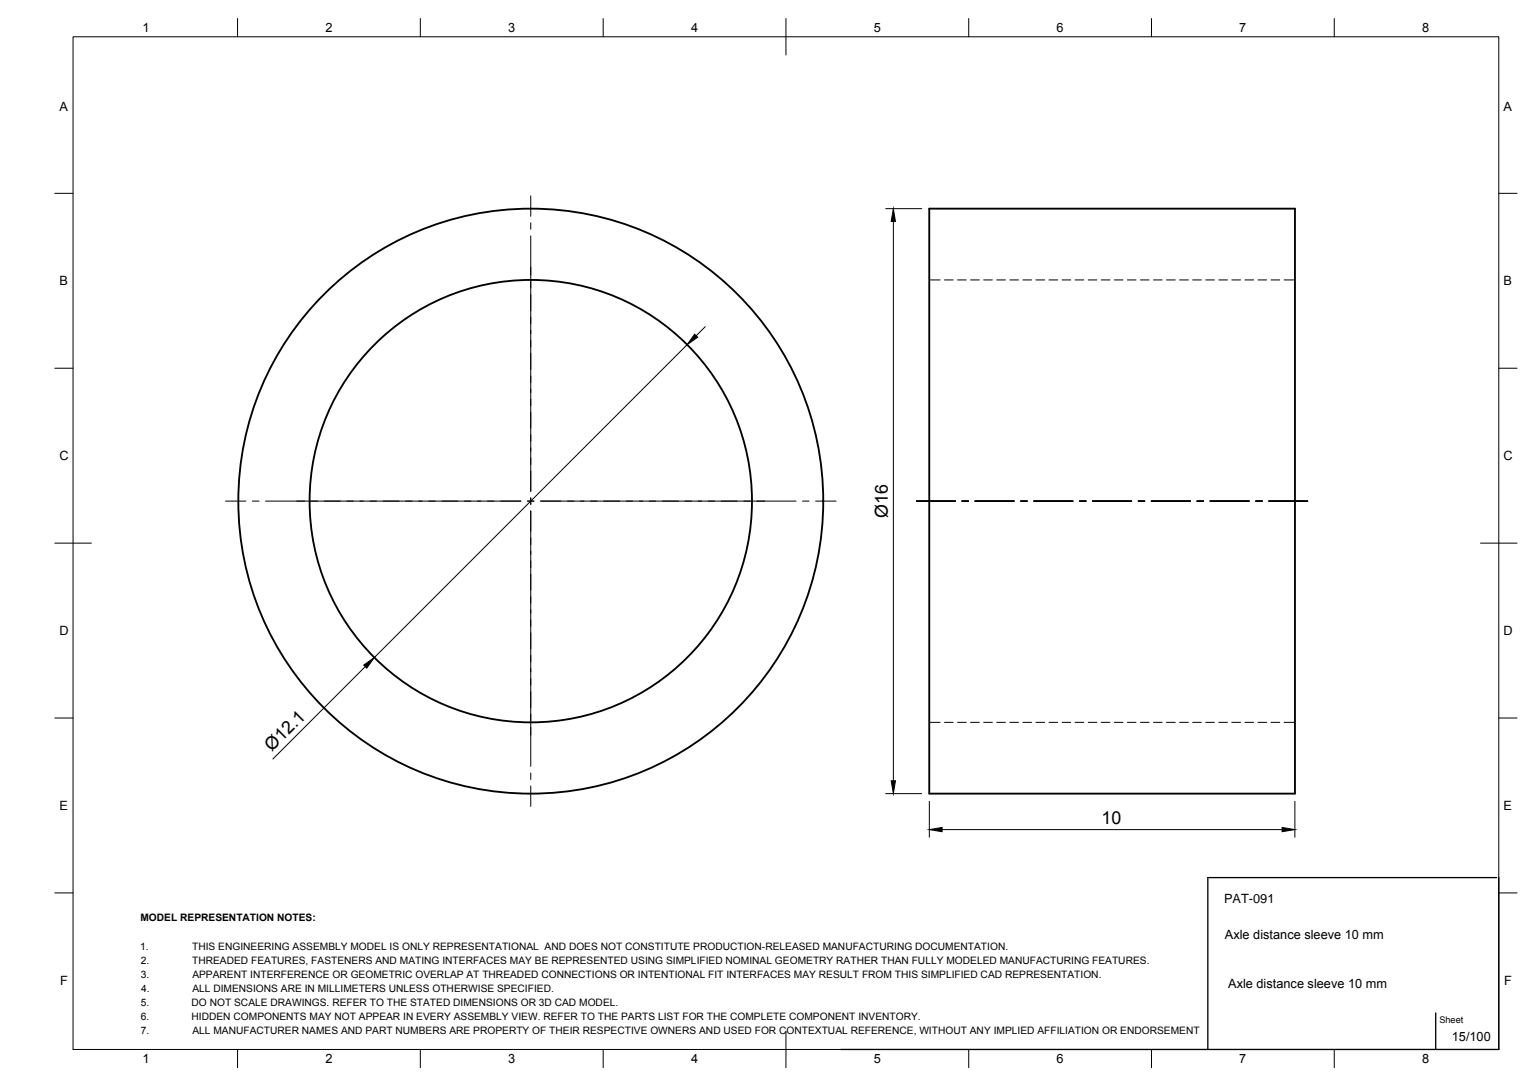
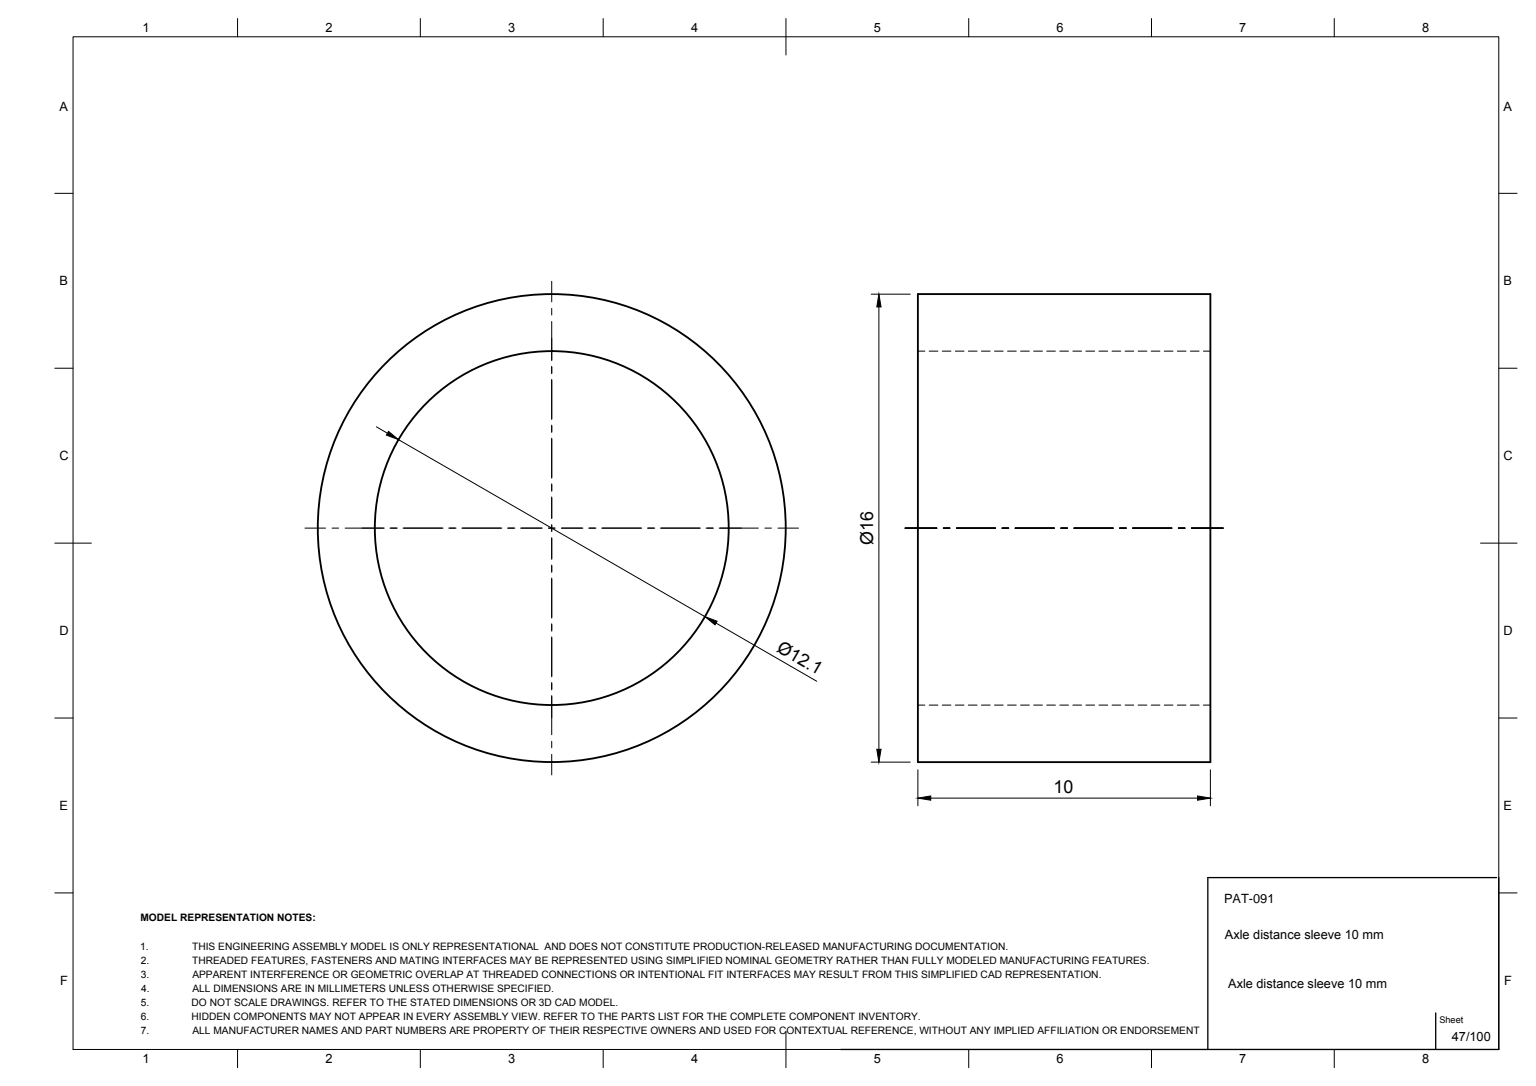
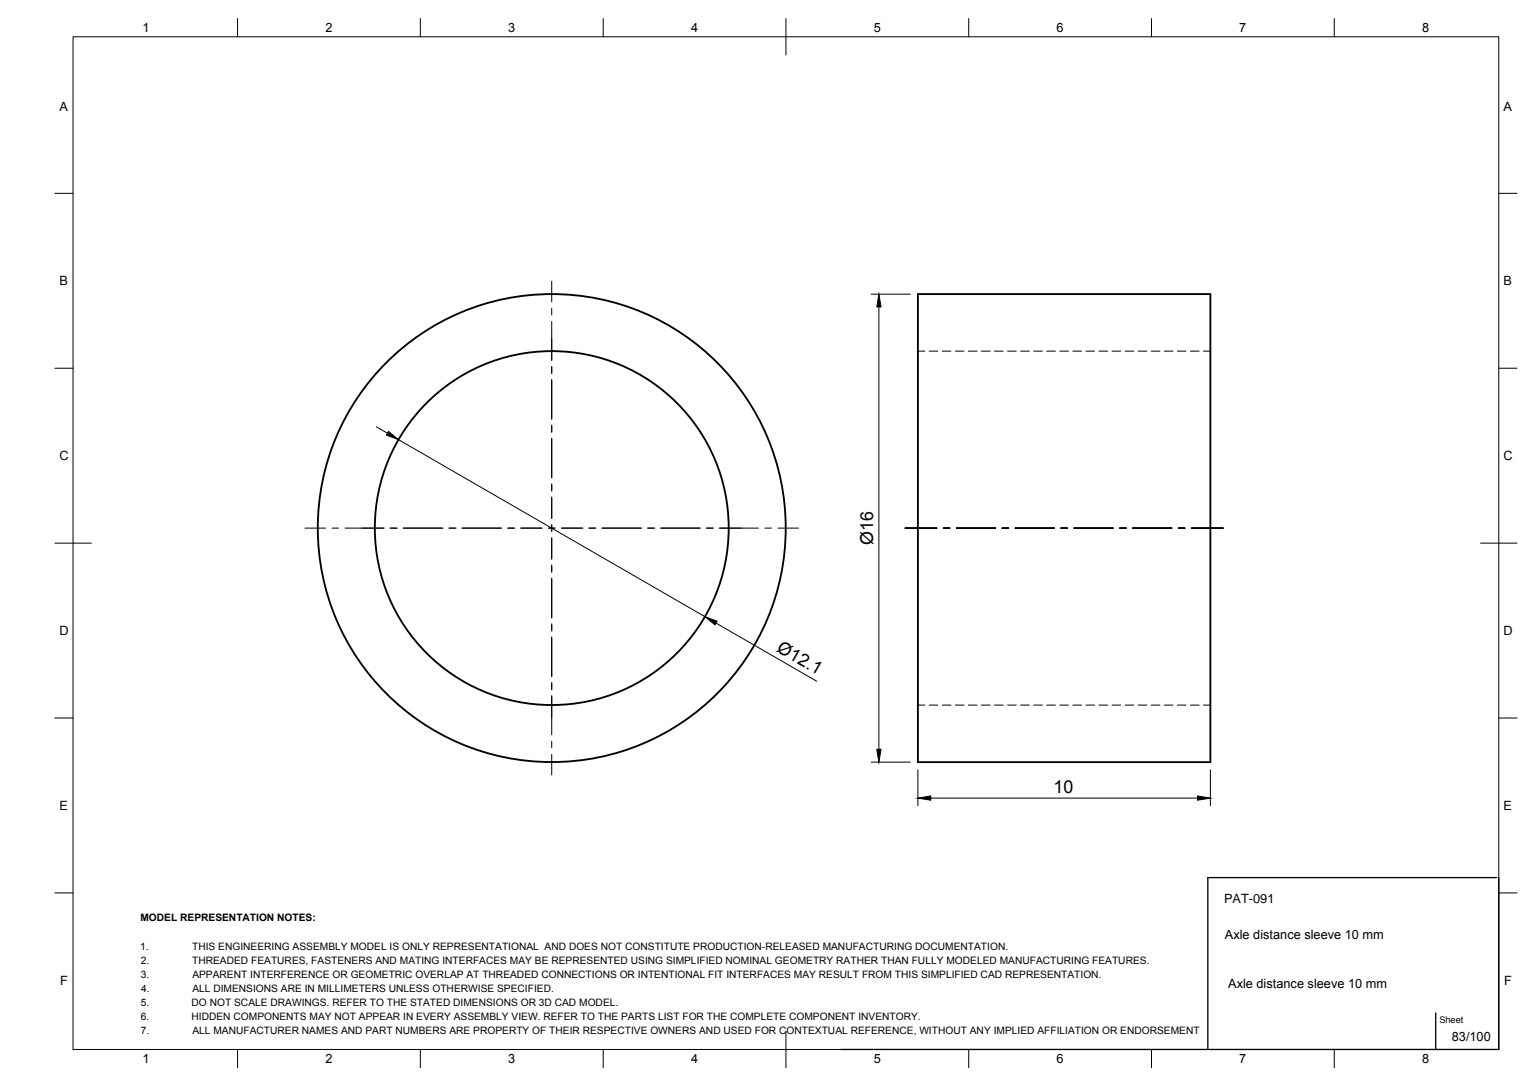
ISO-10303-21;
HEADER;
/* Generated by software containing ST-Developer
 * from STEP Tools, Inc. (www.steptools.com) 
 */

FILE_DESCRIPTION(
/* description */ ('PAT-091'),
/* implementation_level */ '2;1');

FILE_NAME(
/* name */ 'Axle distance sleeve 10 mm.step',
/* time_stamp */ '2026-10-27T15:34:44-07:00',
/* author */ (''),
/* organization */ (''),
/* preprocessor_version */ 'ST-DEVELOPER v20.2',
/* originating_system */ 'Autodesk Translation Framework v15.17.0.0',
/* authorisation */ '');

FILE_SCHEMA (('AUTOMOTIVE_DESIGN { 1 0 10303 214 3 1 1 }'));
ENDSEC;

DATA;
#10=MECHANICAL_DESIGN_GEOMETRIC_PRESENTATION_REPRESENTATION('',(#986),#25100);
#766=SHAPE_REPRESENTATION_RELATIONSHIP('SRR','None',#25527,#876);
#876=ADVANCED_BREP_SHAPE_REPRESENTATION('',(#1110),#24997);
#986=STYLED_ITEM('',(#26191),#1110);
#1110=MANIFOLD_SOLID_BREP('Body1',#13263);
#1329=FACE_BOUND('',#3132,.T.);
#1330=FACE_BOUND('',#3134,.T.);
#1704=PLANE('',#14883);
#1705=PLANE('',#14884);
#2197=FACE_OUTER_BOUND('',#3129,.T.);
#2198=FACE_OUTER_BOUND('',#3130,.T.);
#2199=FACE_OUTER_BOUND('',#3131,.T.);
#2200=FACE_OUTER_BOUND('',#3133,.T.);
#3129=EDGE_LOOP('',(#9560,#9561,#9562,#9563));
#3130=EDGE_LOOP('',(#9564,#9565,#9566,#9567));
#3131=EDGE_LOOP('',(#9568));
#3132=EDGE_LOOP('',(#9569));
#3133=EDGE_LOOP('',(#9570));
#3134=EDGE_LOOP('',(#9571));
#4278=LINE('',#21620,#5018);
#4279=LINE('',#21626,#5019);
#5018=VECTOR('',#17210,0.605);
#5019=VECTOR('',#17217,0.8);
#5744=CIRCLE('',#14878,0.605);
#5745=CIRCLE('',#14879,0.605);
#5746=CIRCLE('',#14881,0.8);
#5747=CIRCLE('',#14882,0.8);
#6579=VERTEX_POINT('',#21617);
#6580=VERTEX_POINT('',#21619);
#6581=VERTEX_POINT('',#21623);
#6582=VERTEX_POINT('',#21625);
#7715=EDGE_CURVE('',#6579,#6579,#5744,.T.);
#7716=EDGE_CURVE('',#6579,#6580,#4278,.T.);
#7717=EDGE_CURVE('',#6580,#6580,#5745,.T.);
#7718=EDGE_CURVE('',#6581,#6581,#5746,.T.);
#7719=EDGE_CURVE('',#6581,#6582,#4279,.T.);
#7720=EDGE_CURVE('',#6582,#6582,#5747,.T.);
#9560=ORIENTED_EDGE('',*,*,#7715,.F.);
#9561=ORIENTED_EDGE('',*,*,#7716,.T.);
#9562=ORIENTED_EDGE('',*,*,#7717,.T.);
#9563=ORIENTED_EDGE('',*,*,#7716,.F.);
#9564=ORIENTED_EDGE('',*,*,#7718,.F.);
#9565=ORIENTED_EDGE('',*,*,#7719,.T.);
#9566=ORIENTED_EDGE('',*,*,#7720,.T.);
#9567=ORIENTED_EDGE('',*,*,#7719,.F.);
#9568=ORIENTED_EDGE('',*,*,#7718,.T.);
#9569=ORIENTED_EDGE('',*,*,#7715,.T.);
#9570=ORIENTED_EDGE('',*,*,#7720,.F.);
#9571=ORIENTED_EDGE('',*,*,#7717,.F.);
#12144=CYLINDRICAL_SURFACE('',#14877,0.605);
#12145=CYLINDRICAL_SURFACE('',#14880,0.8);
#12564=ADVANCED_FACE('',(#2197),#12144,.F.);
#12565=ADVANCED_FACE('',(#2198),#12145,.T.);
#12566=ADVANCED_FACE('',(#2199,#1329),#1704,.T.);
#12567=ADVANCED_FACE('',(#2200,#1330),#1705,.F.);
#13263=CLOSED_SHELL('',(#12564,#12565,#12566,#12567));
#14876=AXIS2_PLACEMENT_3D('',#21615,#17204,#17205);
#14877=AXIS2_PLACEMENT_3D('',#21616,#17206,#17207);
#14878=AXIS2_PLACEMENT_3D('',#21618,#17208,#17209);
#14879=AXIS2_PLACEMENT_3D('',#21621,#17211,#17212);
#14880=AXIS2_PLACEMENT_3D('',#21622,#17213,#17214);
#14881=AXIS2_PLACEMENT_3D('',#21624,#17215,#17216);
#14882=AXIS2_PLACEMENT_3D('',#21627,#17218,#17219);
#14883=AXIS2_PLACEMENT_3D('',#21628,#17220,#17221);
#14884=AXIS2_PLACEMENT_3D('',#21629,#17222,#17223);
#17204=DIRECTION('axis',(0.,0.,1.));
#17205=DIRECTION('refdir',(1.,0.,0.));
#17206=DIRECTION('center_axis',(0.,1.,0.));
#17207=DIRECTION('ref_axis',(1.,0.,0.));
#17208=DIRECTION('center_axis',(0.,-1.,0.));
#17209=DIRECTION('ref_axis',(1.,0.,0.));
#17210=DIRECTION('',(0.,-1.,0.));
#17211=DIRECTION('center_axis',(0.,-1.,0.));
#17212=DIRECTION('ref_axis',(1.,0.,0.));
#17213=DIRECTION('center_axis',(0.,1.,0.));
#17214=DIRECTION('ref_axis',(1.,0.,0.));
#17215=DIRECTION('center_axis',(0.,1.,0.));
#17216=DIRECTION('ref_axis',(1.,0.,0.));
#17217=DIRECTION('',(0.,-1.,0.));
#17218=DIRECTION('center_axis',(0.,1.,0.));
#17219=DIRECTION('ref_axis',(1.,0.,0.));
#17220=DIRECTION('center_axis',(0.,1.,0.));
#17221=DIRECTION('ref_axis',(1.,0.,0.));
#17222=DIRECTION('center_axis',(0.,1.,0.));
#17223=DIRECTION('ref_axis',(1.,0.,0.));
#21615=CARTESIAN_POINT('',(0.,0.,0.));
#21616=CARTESIAN_POINT('Origin',(0.,-6.,3.));
#21617=CARTESIAN_POINT('',(-0.605,-5.,3.));
#21618=CARTESIAN_POINT('Origin',(0.,-5.,3.));
#21619=CARTESIAN_POINT('',(-0.605,-6.,3.));
#21620=CARTESIAN_POINT('',(-0.605,-6.,3.));
#21621=CARTESIAN_POINT('Origin',(0.,-6.,3.));
#21622=CARTESIAN_POINT('Origin',(0.,-6.,3.));
#21623=CARTESIAN_POINT('',(-0.8,-5.,3.));
#21624=CARTESIAN_POINT('Origin',(0.,-5.,3.));
#21625=CARTESIAN_POINT('',(-0.8,-6.,3.));
#21626=CARTESIAN_POINT('',(-0.8,-6.,3.));
#21627=CARTESIAN_POINT('Origin',(0.,-6.,3.));
#21628=CARTESIAN_POINT('Origin',(0.,-5.,3.));
#21629=CARTESIAN_POINT('Origin',(0.,-6.,3.));
#24876=UNCERTAINTY_MEASURE_WITH_UNIT(LENGTH_MEASURE(0.001),#25101,
'DISTANCE_ACCURACY_VALUE',
'Maximum model space distance between geometric entities at asserted c
onnectivities');
#24979=UNCERTAINTY_MEASURE_WITH_UNIT(LENGTH_MEASURE(0.001),#25101,
'DISTANCE_ACCURACY_VALUE',
'Maximum model space distance between geometric entities at asserted c
onnectivities');
#24997=(
GEOMETRIC_REPRESENTATION_CONTEXT(3)
GLOBAL_UNCERTAINTY_ASSIGNED_CONTEXT((#24876))
GLOBAL_UNIT_ASSIGNED_CONTEXT((#25101,#25103,#25104))
REPRESENTATION_CONTEXT('','3D')
);
#25100=(
GEOMETRIC_REPRESENTATION_CONTEXT(3)
GLOBAL_UNCERTAINTY_ASSIGNED_CONTEXT((#24979))
GLOBAL_UNIT_ASSIGNED_CONTEXT((#25101,#25103,#25104))
REPRESENTATION_CONTEXT('','3D')
);
#25101=(
LENGTH_UNIT()
NAMED_UNIT(*)
SI_UNIT(.CENTI.,.METRE.)
);
#25103=(
NAMED_UNIT(*)
PLANE_ANGLE_UNIT()
SI_UNIT($,.RADIAN.)
);
#25104=(
NAMED_UNIT(*)
SI_UNIT($,.STERADIAN.)
SOLID_ANGLE_UNIT()
);
#25122=SHAPE_DEFINITION_REPRESENTATION(#25242,#25527);
#25242=PRODUCT_DEFINITION_SHAPE('',$,#25648);
#25527=SHAPE_REPRESENTATION('',(#14876),#24997);
#25630=PRODUCT_DEFINITION_CONTEXT('part definition',#25992,'design');
#25648=PRODUCT_DEFINITION('Axle distance sleeve 10 mm',
'Axle distance sleeve 10 mm',#25768,#25630);
#25768=PRODUCT_DEFINITION_FORMATION('',$,#26011);
#25992=APPLICATION_CONTEXT(
'Core Data for Automotive Mechanical Design Process');
#25993=PRODUCT_CONTEXT('part definition',#25992,'mechanical');
#26011=PRODUCT('Axle distance sleeve 10 mm',
'Axle distance sleeve 10 mm','Axle distance sleeve 10 mm',(#25993));
#26185=COLOUR_RGB('Grey',0.48,0.52,0.57);
#26186=FILL_AREA_STYLE_COLOUR('',#26185);
#26187=FILL_AREA_STYLE('',(#26186));
#26188=SURFACE_STYLE_FILL_AREA(#26187);
#26189=SURFACE_SIDE_STYLE('',(#26188));
#26190=SURFACE_STYLE_USAGE(.BOTH.,#26189);
#26191=PRESENTATION_STYLE_ASSIGNMENT((#26190));
ENDSEC;
END-ISO-10303-21;
